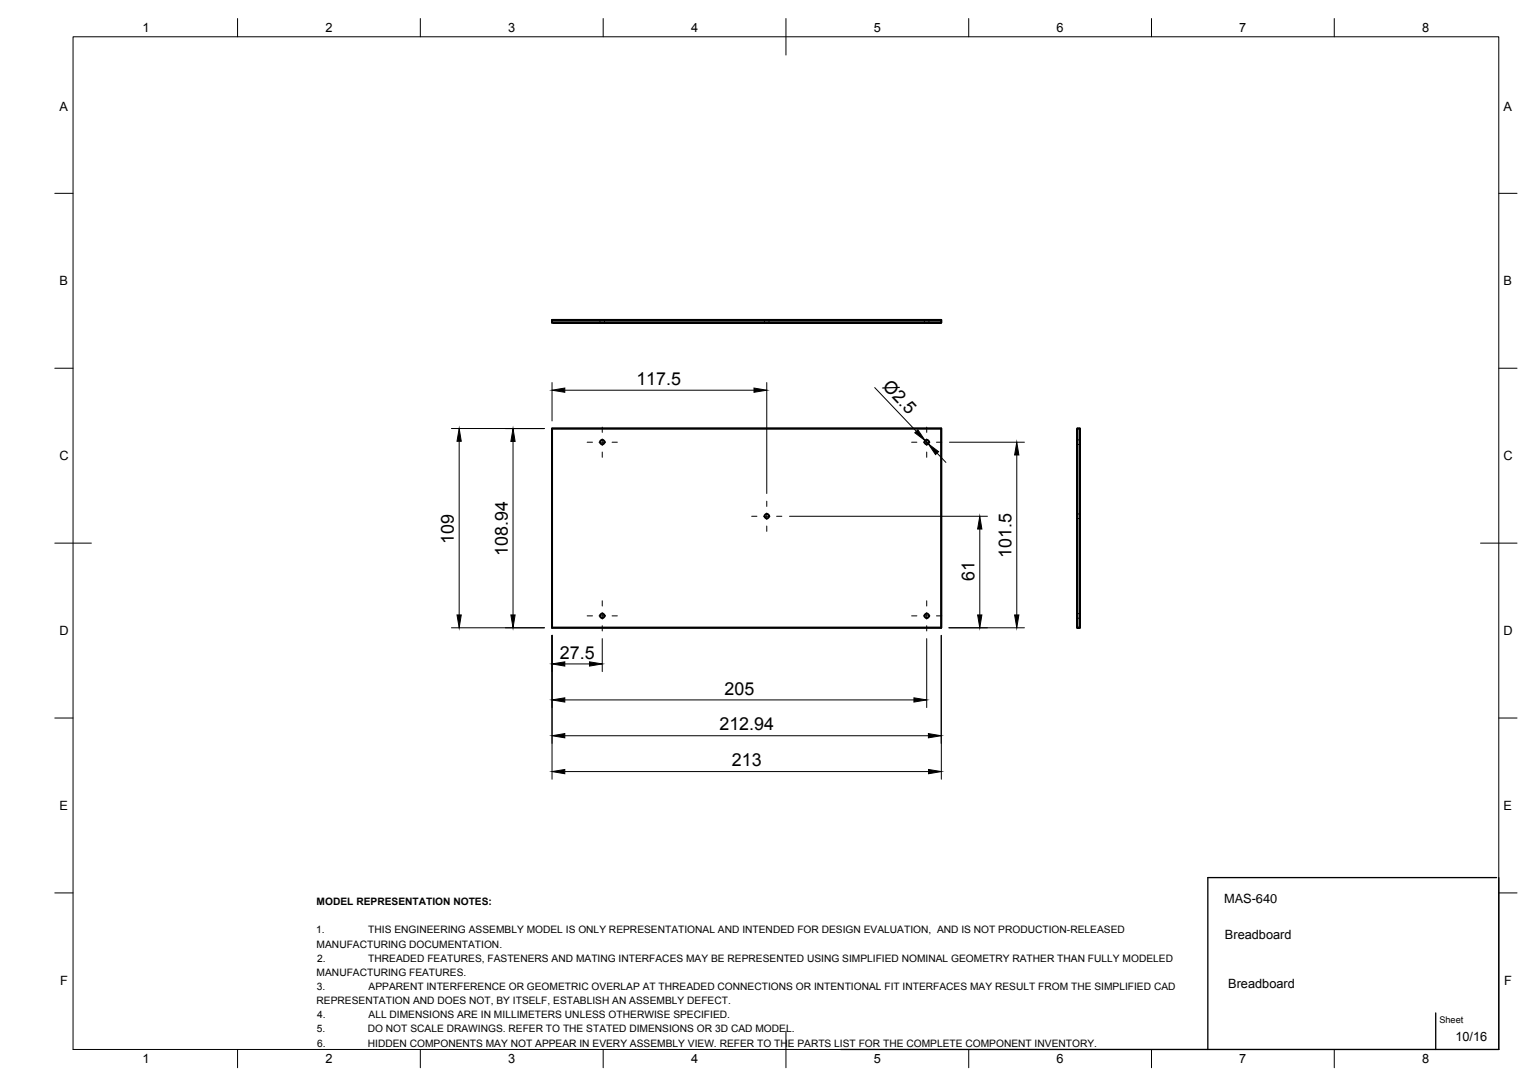
ISO-10303-21;
HEADER;
FILE_DESCRIPTION((''),'2;1');
FILE_NAME('Breadboard.step','2026-10-09T10:33:02-07:00',(''),(''),'','','');
FILE_SCHEMA (('AUTOMOTIVE_DESIGN { 1 0 10303 214 3 1 1 }'));
ENDSEC;
DATA;
#10=MECHANICAL_DESIGN_GEOMETRIC_PRESENTATION_REPRESENTATION('',(#846),#86330);
#822=SHAPE_REPRESENTATION_RELATIONSHIP('SRR','None',#86468,#834) ;
#834=ADVANCED_BREP_SHAPE_REPRESENTATION('',(#858),#86322) ;
#846=STYLED_ITEM('',(#86584),#858) ;
#858=MANIFOLD_SOLID_BREP('Body1',#32645) ;
#1175=FACE_BOUND('',#6134,.T.) ;
#1176=FACE_BOUND('',#6135,.T.) ;
#1177=FACE_BOUND('',#6136,.T.) ;
#1178=FACE_BOUND('',#6137,.T.) ;
#1179=FACE_BOUND('',#6138,.T.) ;
#1180=FACE_BOUND('',#6140,.T.) ;
#1181=FACE_BOUND('',#6141,.T.) ;
#1182=FACE_BOUND('',#6142,.T.) ;
#1183=FACE_BOUND('',#6143,.T.) ;
#1184=FACE_BOUND('',#6144,.T.) ;
#2229=PLANE('',#36344) ;
#2230=PLANE('',#36345) ;
#2231=PLANE('',#36346) ;
#2232=PLANE('',#36347) ;
#2233=PLANE('',#36348) ;
#2234=PLANE('',#36349) ;
#2235=PLANE('',#36350) ;
#2236=PLANE('',#36351) ;
#2237=PLANE('',#36352) ;
#2238=PLANE('',#36353) ;
#2239=PLANE('',#36354) ;
#2240=PLANE('',#36355) ;
#2241=PLANE('',#36356) ;
#2242=PLANE('',#36362) ;
#2243=PLANE('',#36368) ;
#2244=PLANE('',#36369) ;
#2245=PLANE('',#36370) ;
#2246=PLANE('',#36371) ;
#4058=FACE_OUTER_BOUND('',#6121,.T.) ;
#4059=FACE_OUTER_BOUND('',#6122,.T.) ;
#4060=FACE_OUTER_BOUND('',#6123,.T.) ;
#4061=FACE_OUTER_BOUND('',#6124,.T.) ;
#4062=FACE_OUTER_BOUND('',#6125,.T.) ;
#4063=FACE_OUTER_BOUND('',#6126,.T.) ;
#4064=FACE_OUTER_BOUND('',#6127,.T.) ;
#4065=FACE_OUTER_BOUND('',#6128,.T.) ;
#4066=FACE_OUTER_BOUND('',#6129,.T.) ;
#4067=FACE_OUTER_BOUND('',#6130,.T.) ;
#4068=FACE_OUTER_BOUND('',#6131,.T.) ;
#4069=FACE_OUTER_BOUND('',#6132,.T.) ;
#4070=FACE_OUTER_BOUND('',#6133,.T.) ;
#4071=FACE_OUTER_BOUND('',#6139,.T.) ;
#4072=FACE_OUTER_BOUND('',#6145,.T.) ;
#4073=FACE_OUTER_BOUND('',#6146,.T.) ;
#4074=FACE_OUTER_BOUND('',#6147,.T.) ;
#4075=FACE_OUTER_BOUND('',#6148,.T.) ;
#4076=FACE_OUTER_BOUND('',#6149,.T.) ;
#4077=FACE_OUTER_BOUND('',#6150,.T.) ;
#4078=FACE_OUTER_BOUND('',#6151,.T.) ;
#4079=FACE_OUTER_BOUND('',#6152,.T.) ;
#4080=FACE_OUTER_BOUND('',#6153,.T.) ;
#6121=EDGE_LOOP('',(#29412,#29413,#29414,#29415,#29416,#29417)) ;
#6122=EDGE_LOOP('',(#29418,#29419,#29420,#29421,#29422,#29423)) ;
#6123=EDGE_LOOP('',(#29424,#29425,#29426,#29427,#29428,#29429)) ;
#6124=EDGE_LOOP('',(#29430,#29431,#29432,#29433)) ;
#6125=EDGE_LOOP('',(#29434,#29435,#29436,#29437,#29438,#29439)) ;
#6126=EDGE_LOOP('',(#29440,#29441,#29442,#29443,#29444,#29445)) ;
#6127=EDGE_LOOP('',(#29446,#29447,#29448,#29449,#29450,#29451)) ;
#6128=EDGE_LOOP('',(#29452,#29453,#29454,#29455,#29456,#29457)) ;
#6129=EDGE_LOOP('',(#29458,#29459,#29460,#29461)) ;
#6130=EDGE_LOOP('',(#29462,#29463,#29464,#29465,#29466,#29467)) ;
#6131=EDGE_LOOP('',(#29468,#29469,#29470,#29471,#29472,#29473)) ;
#6132=EDGE_LOOP('',(#29474,#29475,#29476,#29477)) ;
#6133=EDGE_LOOP('',(#29478,#29479,#29480,#29481)) ;
#6134=EDGE_LOOP('',(#29482)) ;
#6135=EDGE_LOOP('',(#29483)) ;
#6136=EDGE_LOOP('',(#29484)) ;
#6137=EDGE_LOOP('',(#29485)) ;
#6138=EDGE_LOOP('',(#29486)) ;
#6139=EDGE_LOOP('',(#29487,#29488,#29489,#29490)) ;
#6140=EDGE_LOOP('',(#29491)) ;
#6141=EDGE_LOOP('',(#29492)) ;
#6142=EDGE_LOOP('',(#29493)) ;
#6143=EDGE_LOOP('',(#29494)) ;
#6144=EDGE_LOOP('',(#29495)) ;
#6145=EDGE_LOOP('',(#29496,#29497,#29498,#29499,#29500,#29501)) ;
#6146=EDGE_LOOP('',(#29502,#29503,#29504,#29505)) ;
#6147=EDGE_LOOP('',(#29506,#29507,#29508,#29509,#29510,#29511)) ;
#6148=EDGE_LOOP('',(#29512,#29513,#29514,#29515,#29516,#29517)) ;
#6149=EDGE_LOOP('',(#29518,#29519,#29520,#29521)) ;
#6150=EDGE_LOOP('',(#29522,#29523,#29524,#29525)) ;
#6151=EDGE_LOOP('',(#29526,#29527,#29528,#29529)) ;
#6152=EDGE_LOOP('',(#29530,#29531,#29532,#29533)) ;
#6153=EDGE_LOOP('',(#29534,#29535,#29536,#29537)) ;
#8429=LINE('',#81667,#10748) ;
#8430=LINE('',#81669,#10749) ;
#8431=LINE('',#81671,#10750) ;
#8432=LINE('',#81673,#10751) ;
#8433=LINE('',#81675,#10752) ;
#8434=LINE('',#81676,#10753) ;
#8435=LINE('',#81679,#10754) ;
#8436=LINE('',#81681,#10755) ;
#8437=LINE('',#81683,#10756) ;
#8438=LINE('',#81685,#10757) ;
#8439=LINE('',#81686,#10758) ;
#8440=LINE('',#81689,#10759) ;
#8441=LINE('',#81691,#10760) ;
#8442=LINE('',#81693,#10761) ;
#8443=LINE('',#81694,#10762) ;
#8444=LINE('',#81697,#10763) ;
#8445=LINE('',#81698,#10764) ;
#8446=LINE('',#81702,#10765) ;
#8447=LINE('',#81704,#10766) ;
#8448=LINE('',#81705,#10767) ;
#8449=LINE('',#81706,#10768) ;
#8450=LINE('',#81709,#10769) ;
#8451=LINE('',#81711,#10770) ;
#8452=LINE('',#81713,#10771) ;
#8453=LINE('',#81714,#10772) ;
#8454=LINE('',#81718,#10773) ;
#8455=LINE('',#81720,#10774) ;
#8456=LINE('',#81721,#10775) ;
#8457=LINE('',#81723,#10776) ;
#8458=LINE('',#81724,#10777) ;
#8459=LINE('',#81727,#10778) ;
#8460=LINE('',#81728,#10779) ;
#8461=LINE('',#81729,#10780) ;
#8462=LINE('',#81732,#10781) ;
#8463=LINE('',#81733,#10782) ;
#8464=LINE('',#81736,#10783) ;
#8465=LINE('',#81738,#10784) ;
#8466=LINE('',#81740,#10785) ;
#8467=LINE('',#81741,#10786) ;
#8468=LINE('',#81744,#10787) ;
#8469=LINE('',#81745,#10788) ;
#8470=LINE('',#81748,#10789) ;
#8471=LINE('',#81760,#10790) ;
#8472=LINE('',#81773,#10791) ;
#8473=LINE('',#81774,#10792) ;
#8474=LINE('',#81777,#10793) ;
#8475=LINE('',#81778,#10794) ;
#8476=LINE('',#81780,#10795) ;
#8477=LINE('',#81783,#10796) ;
#8478=LINE('',#81785,#10797) ;
#8479=LINE('',#81787,#10798) ;
#8480=LINE('',#81789,#10799) ;
#8481=LINE('',#81791,#10800) ;
#10748=VECTOR('',#45865,10.) ;
#10749=VECTOR('',#45866,10.) ;
#10750=VECTOR('',#45867,10.) ;
#10751=VECTOR('',#45868,9.99999999999998) ;
#10752=VECTOR('',#45869,10.) ;
#10753=VECTOR('',#45870,10.) ;
#10754=VECTOR('',#45873,10.) ;
#10755=VECTOR('',#45874,10.) ;
#10756=VECTOR('',#45875,10.) ;
#10757=VECTOR('',#45876,10.) ;
#10758=VECTOR('',#45877,10.) ;
#10759=VECTOR('',#45880,10.) ;
#10760=VECTOR('',#45881,10.) ;
#10761=VECTOR('',#45882,10.) ;
#10762=VECTOR('',#45883,10.) ;
#10763=VECTOR('',#45886,10.) ;
#10764=VECTOR('',#45887,10.) ;
#10765=VECTOR('',#45890,10.) ;
#10766=VECTOR('',#45891,10.) ;
#10767=VECTOR('',#45892,10.) ;
#10768=VECTOR('',#45893,10.) ;
#10769=VECTOR('',#45896,10.) ;
#10770=VECTOR('',#45897,10.) ;
#10771=VECTOR('',#45898,10.) ;
#10772=VECTOR('',#45899,10.) ;
#10773=VECTOR('',#45902,10.) ;
#10774=VECTOR('',#45903,10.) ;
#10775=VECTOR('',#45904,10.) ;
#10776=VECTOR('',#45905,10.) ;
#10777=VECTOR('',#45906,10.) ;
#10778=VECTOR('',#45909,10.) ;
#10779=VECTOR('',#45910,10.) ;
#10780=VECTOR('',#45911,10.) ;
#10781=VECTOR('',#45914,10.) ;
#10782=VECTOR('',#45915,10.) ;
#10783=VECTOR('',#45918,10.) ;
#10784=VECTOR('',#45919,10.) ;
#10785=VECTOR('',#45920,10.) ;
#10786=VECTOR('',#45921,10.) ;
#10787=VECTOR('',#45924,10.) ;
#10788=VECTOR('',#45925,10.) ;
#10789=VECTOR('',#45930,10.) ;
#10790=VECTOR('',#45943,10.) ;
#10791=VECTOR('',#45956,10.) ;
#10792=VECTOR('',#45957,10.) ;
#10793=VECTOR('',#45960,10.) ;
#10794=VECTOR('',#45961,10.) ;
#10795=VECTOR('',#45964,10.) ;
#10796=VECTOR('',#45969,1.25) ;
#10797=VECTOR('',#45972,1.25) ;
#10798=VECTOR('',#45975,1.25) ;
#10799=VECTOR('',#45978,1.25) ;
#10800=VECTOR('',#45981,1.25) ;
#12609=CIRCLE('',#36357,1.25) ;
#12610=CIRCLE('',#36358,1.25) ;
#12611=CIRCLE('',#36359,1.25) ;
#12612=CIRCLE('',#36360,1.25) ;
#12613=CIRCLE('',#36361,1.25) ;
#12614=CIRCLE('',#36363,1.25) ;
#12615=CIRCLE('',#36364,1.25) ;
#12616=CIRCLE('',#36365,1.25) ;
#12617=CIRCLE('',#36366,1.25) ;
#12618=CIRCLE('',#36367,1.25) ;
#15418=VERTEX_POINT('',#81665) ;
#15419=VERTEX_POINT('',#81666) ;
#15420=VERTEX_POINT('',#81668) ;
#15421=VERTEX_POINT('',#81670) ;
#15422=VERTEX_POINT('',#81672) ;
#15423=VERTEX_POINT('',#81674) ;
#15424=VERTEX_POINT('',#81678) ;
#15425=VERTEX_POINT('',#81680) ;
#15426=VERTEX_POINT('',#81682) ;
#15427=VERTEX_POINT('',#81684) ;
#15428=VERTEX_POINT('',#81688) ;
#15429=VERTEX_POINT('',#81690) ;
#15430=VERTEX_POINT('',#81692) ;
#15431=VERTEX_POINT('',#81696) ;
#15432=VERTEX_POINT('',#81700) ;
#15433=VERTEX_POINT('',#81701) ;
#15434=VERTEX_POINT('',#81703) ;
#15435=VERTEX_POINT('',#81708) ;
#15436=VERTEX_POINT('',#81710) ;
#15437=VERTEX_POINT('',#81712) ;
#15438=VERTEX_POINT('',#81716) ;
#15439=VERTEX_POINT('',#81717) ;
#15440=VERTEX_POINT('',#81719) ;
#15441=VERTEX_POINT('',#81722) ;
#15442=VERTEX_POINT('',#81726) ;
#15443=VERTEX_POINT('',#81731) ;
#15444=VERTEX_POINT('',#81735) ;
#15445=VERTEX_POINT('',#81737) ;
#15446=VERTEX_POINT('',#81739) ;
#15447=VERTEX_POINT('',#81743) ;
#15448=VERTEX_POINT('',#81749) ;
#15449=VERTEX_POINT('',#81751) ;
#15450=VERTEX_POINT('',#81753) ;
#15451=VERTEX_POINT('',#81755) ;
#15452=VERTEX_POINT('',#81757) ;
#15453=VERTEX_POINT('',#81761) ;
#15454=VERTEX_POINT('',#81763) ;
#15455=VERTEX_POINT('',#81765) ;
#15456=VERTEX_POINT('',#81767) ;
#15457=VERTEX_POINT('',#81769) ;
#15458=VERTEX_POINT('',#81772) ;
#15459=VERTEX_POINT('',#81776) ;
#20112=EDGE_CURVE('',#15418,#15419,#8429,.T.) ;
#20113=EDGE_CURVE('',#15419,#15420,#8430,.T.) ;
#20114=EDGE_CURVE('',#15420,#15421,#8431,.T.) ;
#20115=EDGE_CURVE('',#15421,#15422,#8432,.T.) ;
#20116=EDGE_CURVE('',#15422,#15423,#8433,.T.) ;
#20117=EDGE_CURVE('',#15423,#15418,#8434,.T.) ;
#20118=EDGE_CURVE('',#15424,#15421,#8435,.T.) ;
#20119=EDGE_CURVE('',#15424,#15425,#8436,.T.) ;
#20120=EDGE_CURVE('',#15426,#15425,#8437,.T.) ;
#20121=EDGE_CURVE('',#15427,#15426,#8438,.T.) ;
#20122=EDGE_CURVE('',#15427,#15422,#8439,.T.) ;
#20123=EDGE_CURVE('',#15420,#15428,#8440,.T.) ;
#20124=EDGE_CURVE('',#15429,#15428,#8441,.T.) ;
#20125=EDGE_CURVE('',#15429,#15430,#8442,.T.) ;
#20126=EDGE_CURVE('',#15430,#15424,#8443,.T.) ;
#20127=EDGE_CURVE('',#15431,#15419,#8444,.T.) ;
#20128=EDGE_CURVE('',#15428,#15431,#8445,.T.) ;
#20129=EDGE_CURVE('',#15432,#15433,#8446,.T.) ;
#20130=EDGE_CURVE('',#15433,#15434,#8447,.T.) ;
#20131=EDGE_CURVE('',#15434,#15429,#8448,.T.) ;
#20132=EDGE_CURVE('',#15431,#15432,#8449,.T.) ;
#20133=EDGE_CURVE('',#15434,#15435,#8450,.T.) ;
#20134=EDGE_CURVE('',#15436,#15435,#8451,.T.) ;
#20135=EDGE_CURVE('',#15437,#15436,#8452,.T.) ;
#20136=EDGE_CURVE('',#15437,#15430,#8453,.T.) ;
#20137=EDGE_CURVE('',#15438,#15439,#8454,.T.) ;
#20138=EDGE_CURVE('',#15439,#15440,#8455,.T.) ;
#20139=EDGE_CURVE('',#15440,#15436,#8456,.T.) ;
#20140=EDGE_CURVE('',#15435,#15441,#8457,.T.) ;
#20141=EDGE_CURVE('',#15441,#15438,#8458,.T.) ;
#20142=EDGE_CURVE('',#15440,#15442,#8459,.T.) ;
#20143=EDGE_CURVE('',#15426,#15442,#8460,.T.) ;
#20144=EDGE_CURVE('',#15425,#15437,#8461,.T.) ;
#20145=EDGE_CURVE('',#15443,#15439,#8462,.T.) ;
#20146=EDGE_CURVE('',#15442,#15443,#8463,.T.) ;
#20147=EDGE_CURVE('',#15444,#15438,#8464,.T.) ;
#20148=EDGE_CURVE('',#15444,#15445,#8465,.T.) ;
#20149=EDGE_CURVE('',#15446,#15445,#8466,.T.) ;
#20150=EDGE_CURVE('',#15443,#15446,#8467,.T.) ;
#20151=EDGE_CURVE('',#15446,#15447,#8468,.T.) ;
#20152=EDGE_CURVE('',#15447,#15427,#8469,.T.) ;
#20153=EDGE_CURVE('',#15441,#15433,#8470,.T.) ;
#20154=EDGE_CURVE('',#15448,#15448,#12609,.T.) ;
#20155=EDGE_CURVE('',#15449,#15449,#12610,.T.) ;
#20156=EDGE_CURVE('',#15450,#15450,#12611,.T.) ;
#20157=EDGE_CURVE('',#15451,#15451,#12612,.T.) ;
#20158=EDGE_CURVE('',#15452,#15452,#12613,.T.) ;
#20159=EDGE_CURVE('',#15423,#15447,#8471,.T.) ;
#20160=EDGE_CURVE('',#15453,#15453,#12614,.T.) ;
#20161=EDGE_CURVE('',#15454,#15454,#12615,.T.) ;
#20162=EDGE_CURVE('',#15455,#15455,#12616,.T.) ;
#20163=EDGE_CURVE('',#15456,#15456,#12617,.T.) ;
#20164=EDGE_CURVE('',#15457,#15457,#12618,.T.) ;
#20165=EDGE_CURVE('',#15432,#15458,#8472,.T.) ;
#20166=EDGE_CURVE('',#15458,#15444,#8473,.T.) ;
#20167=EDGE_CURVE('',#15459,#15458,#8474,.T.) ;
#20168=EDGE_CURVE('',#15445,#15459,#8475,.T.) ;
#20169=EDGE_CURVE('',#15459,#15418,#8476,.T.) ;
#20170=EDGE_CURVE('',#15452,#15457,#8477,.T.) ;
#20171=EDGE_CURVE('',#15451,#15456,#8478,.T.) ;
#20172=EDGE_CURVE('',#15450,#15455,#8479,.T.) ;
#20173=EDGE_CURVE('',#15449,#15454,#8480,.T.) ;
#20174=EDGE_CURVE('',#15448,#15453,#8481,.T.) ;
#29412=ORIENTED_EDGE('',*,*,#20112,.T.) ;
#29413=ORIENTED_EDGE('',*,*,#20113,.T.) ;
#29414=ORIENTED_EDGE('',*,*,#20114,.T.) ;
#29415=ORIENTED_EDGE('',*,*,#20115,.T.) ;
#29416=ORIENTED_EDGE('',*,*,#20116,.T.) ;
#29417=ORIENTED_EDGE('',*,*,#20117,.T.) ;
#29418=ORIENTED_EDGE('',*,*,#20115,.F.) ;
#29419=ORIENTED_EDGE('',*,*,#20118,.F.) ;
#29420=ORIENTED_EDGE('',*,*,#20119,.T.) ;
#29421=ORIENTED_EDGE('',*,*,#20120,.F.) ;
#29422=ORIENTED_EDGE('',*,*,#20121,.F.) ;
#29423=ORIENTED_EDGE('',*,*,#20122,.T.) ;
#29424=ORIENTED_EDGE('',*,*,#20114,.F.) ;
#29425=ORIENTED_EDGE('',*,*,#20123,.T.) ;
#29426=ORIENTED_EDGE('',*,*,#20124,.F.) ;
#29427=ORIENTED_EDGE('',*,*,#20125,.T.) ;
#29428=ORIENTED_EDGE('',*,*,#20126,.T.) ;
#29429=ORIENTED_EDGE('',*,*,#20118,.T.) ;
#29430=ORIENTED_EDGE('',*,*,#20113,.F.) ;
#29431=ORIENTED_EDGE('',*,*,#20127,.F.) ;
#29432=ORIENTED_EDGE('',*,*,#20128,.F.) ;
#29433=ORIENTED_EDGE('',*,*,#20123,.F.) ;
#29434=ORIENTED_EDGE('',*,*,#20129,.T.) ;
#29435=ORIENTED_EDGE('',*,*,#20130,.T.) ;
#29436=ORIENTED_EDGE('',*,*,#20131,.T.) ;
#29437=ORIENTED_EDGE('',*,*,#20124,.T.) ;
#29438=ORIENTED_EDGE('',*,*,#20128,.T.) ;
#29439=ORIENTED_EDGE('',*,*,#20132,.T.) ;
#29440=ORIENTED_EDGE('',*,*,#20131,.F.) ;
#29441=ORIENTED_EDGE('',*,*,#20133,.T.) ;
#29442=ORIENTED_EDGE('',*,*,#20134,.F.) ;
#29443=ORIENTED_EDGE('',*,*,#20135,.F.) ;
#29444=ORIENTED_EDGE('',*,*,#20136,.T.) ;
#29445=ORIENTED_EDGE('',*,*,#20125,.F.) ;
#29446=ORIENTED_EDGE('',*,*,#20137,.T.) ;
#29447=ORIENTED_EDGE('',*,*,#20138,.T.) ;
#29448=ORIENTED_EDGE('',*,*,#20139,.T.) ;
#29449=ORIENTED_EDGE('',*,*,#20134,.T.) ;
#29450=ORIENTED_EDGE('',*,*,#20140,.T.) ;
#29451=ORIENTED_EDGE('',*,*,#20141,.T.) ;
#29452=ORIENTED_EDGE('',*,*,#20139,.F.) ;
#29453=ORIENTED_EDGE('',*,*,#20142,.T.) ;
#29454=ORIENTED_EDGE('',*,*,#20143,.F.) ;
#29455=ORIENTED_EDGE('',*,*,#20120,.T.) ;
#29456=ORIENTED_EDGE('',*,*,#20144,.T.) ;
#29457=ORIENTED_EDGE('',*,*,#20135,.T.) ;
#29458=ORIENTED_EDGE('',*,*,#20138,.F.) ;
#29459=ORIENTED_EDGE('',*,*,#20145,.F.) ;
#29460=ORIENTED_EDGE('',*,*,#20146,.F.) ;
#29461=ORIENTED_EDGE('',*,*,#20142,.F.) ;
#29462=ORIENTED_EDGE('',*,*,#20137,.F.) ;
#29463=ORIENTED_EDGE('',*,*,#20147,.F.) ;
#29464=ORIENTED_EDGE('',*,*,#20148,.T.) ;
#29465=ORIENTED_EDGE('',*,*,#20149,.F.) ;
#29466=ORIENTED_EDGE('',*,*,#20150,.F.) ;
#29467=ORIENTED_EDGE('',*,*,#20145,.T.) ;
#29468=ORIENTED_EDGE('',*,*,#20143,.T.) ;
#29469=ORIENTED_EDGE('',*,*,#20146,.T.) ;
#29470=ORIENTED_EDGE('',*,*,#20150,.T.) ;
#29471=ORIENTED_EDGE('',*,*,#20151,.T.) ;
#29472=ORIENTED_EDGE('',*,*,#20152,.T.) ;
#29473=ORIENTED_EDGE('',*,*,#20121,.T.) ;
#29474=ORIENTED_EDGE('',*,*,#20144,.F.) ;
#29475=ORIENTED_EDGE('',*,*,#20119,.F.) ;
#29476=ORIENTED_EDGE('',*,*,#20126,.F.) ;
#29477=ORIENTED_EDGE('',*,*,#20136,.F.) ;
#29478=ORIENTED_EDGE('',*,*,#20130,.F.) ;
#29479=ORIENTED_EDGE('',*,*,#20153,.F.) ;
#29480=ORIENTED_EDGE('',*,*,#20140,.F.) ;
#29481=ORIENTED_EDGE('',*,*,#20133,.F.) ;
#29482=ORIENTED_EDGE('',*,*,#20154,.F.) ;
#29483=ORIENTED_EDGE('',*,*,#20155,.F.) ;
#29484=ORIENTED_EDGE('',*,*,#20156,.F.) ;
#29485=ORIENTED_EDGE('',*,*,#20157,.F.) ;
#29486=ORIENTED_EDGE('',*,*,#20158,.F.) ;
#29487=ORIENTED_EDGE('',*,*,#20116,.F.) ;
#29488=ORIENTED_EDGE('',*,*,#20122,.F.) ;
#29489=ORIENTED_EDGE('',*,*,#20152,.F.) ;
#29490=ORIENTED_EDGE('',*,*,#20159,.F.) ;
#29491=ORIENTED_EDGE('',*,*,#20160,.F.) ;
#29492=ORIENTED_EDGE('',*,*,#20161,.F.) ;
#29493=ORIENTED_EDGE('',*,*,#20162,.F.) ;
#29494=ORIENTED_EDGE('',*,*,#20163,.F.) ;
#29495=ORIENTED_EDGE('',*,*,#20164,.F.) ;
#29496=ORIENTED_EDGE('',*,*,#20129,.F.) ;
#29497=ORIENTED_EDGE('',*,*,#20165,.T.) ;
#29498=ORIENTED_EDGE('',*,*,#20166,.T.) ;
#29499=ORIENTED_EDGE('',*,*,#20147,.T.) ;
#29500=ORIENTED_EDGE('',*,*,#20141,.F.) ;
#29501=ORIENTED_EDGE('',*,*,#20153,.T.) ;
#29502=ORIENTED_EDGE('',*,*,#20166,.F.) ;
#29503=ORIENTED_EDGE('',*,*,#20167,.F.) ;
#29504=ORIENTED_EDGE('',*,*,#20168,.F.) ;
#29505=ORIENTED_EDGE('',*,*,#20148,.F.) ;
#29506=ORIENTED_EDGE('',*,*,#20117,.F.) ;
#29507=ORIENTED_EDGE('',*,*,#20159,.T.) ;
#29508=ORIENTED_EDGE('',*,*,#20151,.F.) ;
#29509=ORIENTED_EDGE('',*,*,#20149,.T.) ;
#29510=ORIENTED_EDGE('',*,*,#20168,.T.) ;
#29511=ORIENTED_EDGE('',*,*,#20169,.T.) ;
#29512=ORIENTED_EDGE('',*,*,#20112,.F.) ;
#29513=ORIENTED_EDGE('',*,*,#20169,.F.) ;
#29514=ORIENTED_EDGE('',*,*,#20167,.T.) ;
#29515=ORIENTED_EDGE('',*,*,#20165,.F.) ;
#29516=ORIENTED_EDGE('',*,*,#20132,.F.) ;
#29517=ORIENTED_EDGE('',*,*,#20127,.T.) ;
#29518=ORIENTED_EDGE('',*,*,#20158,.T.) ;
#29519=ORIENTED_EDGE('',*,*,#20170,.T.) ;
#29520=ORIENTED_EDGE('',*,*,#20164,.T.) ;
#29521=ORIENTED_EDGE('',*,*,#20170,.F.) ;
#29522=ORIENTED_EDGE('',*,*,#20157,.T.) ;
#29523=ORIENTED_EDGE('',*,*,#20171,.T.) ;
#29524=ORIENTED_EDGE('',*,*,#20163,.T.) ;
#29525=ORIENTED_EDGE('',*,*,#20171,.F.) ;
#29526=ORIENTED_EDGE('',*,*,#20156,.T.) ;
#29527=ORIENTED_EDGE('',*,*,#20172,.T.) ;
#29528=ORIENTED_EDGE('',*,*,#20162,.T.) ;
#29529=ORIENTED_EDGE('',*,*,#20172,.F.) ;
#29530=ORIENTED_EDGE('',*,*,#20155,.T.) ;
#29531=ORIENTED_EDGE('',*,*,#20173,.T.) ;
#29532=ORIENTED_EDGE('',*,*,#20161,.T.) ;
#29533=ORIENTED_EDGE('',*,*,#20173,.F.) ;
#29534=ORIENTED_EDGE('',*,*,#20154,.T.) ;
#29535=ORIENTED_EDGE('',*,*,#20174,.T.) ;
#29536=ORIENTED_EDGE('',*,*,#20160,.T.) ;
#29537=ORIENTED_EDGE('',*,*,#20174,.F.) ;
#30707=CYLINDRICAL_SURFACE('',#36372,1.25) ;
#30708=CYLINDRICAL_SURFACE('',#36373,1.25) ;
#30709=CYLINDRICAL_SURFACE('',#36374,1.25) ;
#30710=CYLINDRICAL_SURFACE('',#36375,1.25) ;
#30711=CYLINDRICAL_SURFACE('',#36376,1.25) ;
#32537=ADVANCED_FACE('',(#4058),#2229,.T.) ;
#32538=ADVANCED_FACE('',(#4059),#2230,.T.) ;
#32539=ADVANCED_FACE('',(#4060),#2231,.T.) ;
#32540=ADVANCED_FACE('',(#4061),#2232,.T.) ;
#32541=ADVANCED_FACE('',(#4062),#2233,.T.) ;
#32542=ADVANCED_FACE('',(#4063),#2234,.T.) ;
#32543=ADVANCED_FACE('',(#4064),#2235,.T.) ;
#32544=ADVANCED_FACE('',(#4065),#2236,.T.) ;
#32545=ADVANCED_FACE('',(#4066),#2237,.T.) ;
#32546=ADVANCED_FACE('',(#4067),#2238,.T.) ;
#32547=ADVANCED_FACE('',(#4068),#2239,.T.) ;
#32548=ADVANCED_FACE('',(#4069),#2240,.T.) ;
#32549=ADVANCED_FACE('',(#4070,#1175,#1176,#1177,#1178,#1179),#2241,.T.) ;
#32550=ADVANCED_FACE('',(#4071,#1180,#1181,#1182,#1183,#1184),#2242,.T.) ;
#32551=ADVANCED_FACE('',(#4072),#2243,.T.) ;
#32552=ADVANCED_FACE('',(#4073),#2244,.F.) ;
#32553=ADVANCED_FACE('',(#4074),#2245,.T.) ;
#32554=ADVANCED_FACE('',(#4075),#2246,.T.) ;
#32555=ADVANCED_FACE('',(#4076),#30707,.F.) ;
#32556=ADVANCED_FACE('',(#4077),#30708,.F.) ;
#32557=ADVANCED_FACE('',(#4078),#30709,.F.) ;
#32558=ADVANCED_FACE('',(#4079),#30710,.F.) ;
#32559=ADVANCED_FACE('',(#4080),#30711,.F.) ;
#32645=CLOSED_SHELL('',(#32537,#32538,#32539,#32540,#32541,#32542,#32543,
#32544,#32545,#32546,#32547,#32548,#32549,#32550,#32551,#32552,#32553,#32554,
#32555,#32556,#32557,#32558,#32559)) ;
#36343=AXIS2_PLACEMENT_3D('',#81663,#45861,#45862) ;
#36344=AXIS2_PLACEMENT_3D('',#81664,#45863,#45864) ;
#36345=AXIS2_PLACEMENT_3D('',#81677,#45871,#45872) ;
#36346=AXIS2_PLACEMENT_3D('',#81687,#45878,#45879) ;
#36347=AXIS2_PLACEMENT_3D('',#81695,#45884,#45885) ;
#36348=AXIS2_PLACEMENT_3D('',#81699,#45888,#45889) ;
#36349=AXIS2_PLACEMENT_3D('',#81707,#45894,#45895) ;
#36350=AXIS2_PLACEMENT_3D('',#81715,#45900,#45901) ;
#36351=AXIS2_PLACEMENT_3D('',#81725,#45907,#45908) ;
#36352=AXIS2_PLACEMENT_3D('',#81730,#45912,#45913) ;
#36353=AXIS2_PLACEMENT_3D('',#81734,#45916,#45917) ;
#36354=AXIS2_PLACEMENT_3D('',#81742,#45922,#45923) ;
#36355=AXIS2_PLACEMENT_3D('',#81746,#45926,#45927) ;
#36356=AXIS2_PLACEMENT_3D('',#81747,#45928,#45929) ;
#36357=AXIS2_PLACEMENT_3D('',#81750,#45931,#45932) ;
#36358=AXIS2_PLACEMENT_3D('',#81752,#45933,#45934) ;
#36359=AXIS2_PLACEMENT_3D('',#81754,#45935,#45936) ;
#36360=AXIS2_PLACEMENT_3D('',#81756,#45937,#45938) ;
#36361=AXIS2_PLACEMENT_3D('',#81758,#45939,#45940) ;
#36362=AXIS2_PLACEMENT_3D('',#81759,#45941,#45942) ;
#36363=AXIS2_PLACEMENT_3D('',#81762,#45944,#45945) ;
#36364=AXIS2_PLACEMENT_3D('',#81764,#45946,#45947) ;
#36365=AXIS2_PLACEMENT_3D('',#81766,#45948,#45949) ;
#36366=AXIS2_PLACEMENT_3D('',#81768,#45950,#45951) ;
#36367=AXIS2_PLACEMENT_3D('',#81770,#45952,#45953) ;
#36368=AXIS2_PLACEMENT_3D('',#81771,#45954,#45955) ;
#36369=AXIS2_PLACEMENT_3D('',#81775,#45958,#45959) ;
#36370=AXIS2_PLACEMENT_3D('',#81779,#45962,#45963) ;
#36371=AXIS2_PLACEMENT_3D('',#81781,#45965,#45966) ;
#36372=AXIS2_PLACEMENT_3D('',#81782,#45967,#45968) ;
#36373=AXIS2_PLACEMENT_3D('',#81784,#45970,#45971) ;
#36374=AXIS2_PLACEMENT_3D('',#81786,#45973,#45974) ;
#36375=AXIS2_PLACEMENT_3D('',#81788,#45976,#45977) ;
#36376=AXIS2_PLACEMENT_3D('',#81790,#45979,#45980) ;
#45861=DIRECTION('axis',(0.,0.,1.)) ;
#45862=DIRECTION('refdir',(1.,0.,0.)) ;
#45863=DIRECTION('center_axis',(-3.21164817626321E-14,0.707106781183433,
-0.707106781189663)) ;
#45864=DIRECTION('ref_axis',(-1.,4.59435859315612E-29,4.54195640842224E-14)) ;
#45865=DIRECTION('',(-0.577350269185717,-0.577350269194137,-0.577350269189023)) ;
#45866=DIRECTION('',(-1.,-4.54195640846222E-14,4.43134223659454E-28)) ;
#45867=DIRECTION('',(-0.577350269188067,0.577350269192936,0.577350269187875)) ;
#45868=DIRECTION('',(0.57735026919122,0.577350269191385,0.577350269186272)) ;
#45869=DIRECTION('',(1.,4.54195640846222E-14,-4.43134223659454E-28)) ;
#45870=DIRECTION('',(0.577350269190983,-0.577350269191477,-0.577350269186417)) ;
#45871=DIRECTION('center_axis',(-0.707106781186648,0.707106781186447,-2.17344707950985E-15)) ;
#45872=DIRECTION('ref_axis',(-3.07371833694259E-15,-1.89978378844695E-30,
1.)) ;
#45873=DIRECTION('',(0.577350269189617,0.577350269189779,-0.577350269189481)) ;
#45874=DIRECTION('',(3.03527276676558E-28,3.07371833694377E-15,1.)) ;
#45875=DIRECTION('',(-0.577350269189562,-0.577350269189728,-0.577350269189587)) ;
#45876=DIRECTION('',(-0.577350269187503,-0.577350269187665,0.57735026919371)) ;
#45877=DIRECTION('',(-3.03527276676558E-28,-3.07371833694377E-15,-1.)) ;
#45878=DIRECTION('center_axis',(-0.707106781186447,-3.42899288422795E-14,
-0.707106781186648)) ;
#45879=DIRECTION('ref_axis',(-0.707106781186648,-5.24209240922293E-31,0.707106781186447)) ;
#45880=DIRECTION('',(4.54195640846222E-14,-1.,3.07371833694377E-15)) ;
#45881=DIRECTION('',(0.577350269189872,0.57735026918927,-0.577350269189736)) ;
#45882=DIRECTION('',(-0.577350269189744,0.577350269189582,0.577350269189552)) ;
#45883=DIRECTION('',(-4.54195640846222E-14,1.,-3.07371833694377E-15)) ;
#45884=DIRECTION('center_axis',(-3.03527276676558E-28,-3.07371833694377E-15,
-1.)) ;
#45885=DIRECTION('ref_axis',(-4.54195640846222E-14,1.,-3.07371833694377E-15)) ;
#45886=DIRECTION('',(-4.54195640846222E-14,1.,-3.07371833694377E-15)) ;
#45887=DIRECTION('',(1.,4.54195640846222E-14,-4.43134223659454E-28)) ;
#45888=DIRECTION('center_axis',(3.21164817627867E-14,-0.707106781186849,
-0.707106781186246)) ;
#45889=DIRECTION('ref_axis',(-1.,1.22805031005106E-29,-4.54195640846605E-14)) ;
#45890=DIRECTION('',(-0.577350269186846,-0.577350269190783,0.577350269191249)) ;
#45891=DIRECTION('',(-1.,-4.54195640846222E-14,4.43134223659454E-28)) ;
#45892=DIRECTION('',(-0.577350269189563,0.577350269189398,-0.577350269189916)) ;
#45893=DIRECTION('',(0.577350269187627,-0.577350269190366,0.577350269190884)) ;
#45894=DIRECTION('center_axis',(-0.707106781186447,-0.707106781186648,2.1734470795109E-15)) ;
#45895=DIRECTION('ref_axis',(3.07371833694495E-15,-2.57298801481783E-30,
1.)) ;
#45896=DIRECTION('',(3.03527276676558E-28,3.07371833694377E-15,1.)) ;
#45897=DIRECTION('',(0.577350269189561,-0.577350269189399,-0.577350269189917)) ;
#45898=DIRECTION('',(0.577350269189689,-0.577350269189523,0.577350269189665)) ;
#45899=DIRECTION('',(-3.03527276676558E-28,-3.07371833694377E-15,-1.)) ;
#45900=DIRECTION('center_axis',(3.21164817627873E-14,-0.707106781186849,
0.707106781186246)) ;
#45901=DIRECTION('ref_axis',(1.,-5.21959547942856E-29,-4.54195640846614E-14)) ;
#45902=DIRECTION('',(-0.577350269188176,0.577350269190091,0.57735026919061)) ;
#45903=DIRECTION('',(-1.,-4.54195640846222E-14,4.43134223659454E-28)) ;
#45904=DIRECTION('',(-0.577350269189765,-0.577350269189323,-0.577350269189789)) ;
#45905=DIRECTION('',(1.,4.54195640846222E-14,-4.43134223659454E-28)) ;
#45906=DIRECTION('',(0.577350269186844,0.577350269190784,0.57735026919125)) ;
#45907=DIRECTION('center_axis',(-0.707106781186548,-2.9943034683263E-14,
0.707106781186548)) ;
#45908=DIRECTION('ref_axis',(0.707106781186548,4.34801313340064E-31,0.707106781186548)) ;
#45909=DIRECTION('',(-4.54195640846222E-14,1.,-3.07371833694377E-15)) ;
#45910=DIRECTION('',(0.577350269191675,-0.577350269185553,0.57735026919165)) ;
#45911=DIRECTION('',(4.54195640846222E-14,-1.,3.07371833694377E-15)) ;
#45912=DIRECTION('center_axis',(3.03527276676558E-28,3.07371833694377E-15,
1.)) ;
#45913=DIRECTION('ref_axis',(4.54195640846222E-14,-1.,3.07371833694377E-15)) ;
#45914=DIRECTION('',(4.54195640846222E-14,-1.,3.07371833694377E-15)) ;
#45915=DIRECTION('',(1.,4.54195640846222E-14,-4.43134223659454E-28)) ;
#45916=DIRECTION('center_axis',(0.707106781188055,3.42899288423475E-14,
0.70710678118504)) ;
#45917=DIRECTION('ref_axis',(0.70710678118504,-2.67373424278474E-31,-0.707106781188055)) ;
#45918=DIRECTION('',(-0.577350269187484,-0.57735026919142,0.577350269189973)) ;
#45919=DIRECTION('',(-4.54195640846222E-14,1.,-3.07371833694377E-15)) ;
#45920=DIRECTION('',(0.57735026918865,-0.577350269189144,-0.577350269191083)) ;
#45921=DIRECTION('',(0.577350269189981,0.577350269186425,-0.577350269192471)) ;
#45922=DIRECTION('center_axis',(-3.21164817629419E-14,0.707106781190265,
0.70710678118283)) ;
#45923=DIRECTION('ref_axis',(1.,-2.00665671353E-30,4.54195640850994E-14)) ;
#45924=DIRECTION('',(-0.577350269187266,0.577350269187757,-0.577350269193854)) ;
#45925=DIRECTION('',(-1.,-4.54195640846222E-14,4.43134223659454E-28)) ;
#45926=DIRECTION('center_axis',(-1.,-4.54195640846222E-14,4.43134223659454E-28)) ;
#45927=DIRECTION('ref_axis',(4.54195640846222E-14,-1.,3.07371833694377E-15)) ;
#45928=DIRECTION('center_axis',(4.54195640846222E-14,-1.,3.07371833694377E-15)) ;
#45929=DIRECTION('ref_axis',(-3.03527276676558E-28,-3.07371833694377E-15,
-1.)) ;
#45930=DIRECTION('',(-6.99265107823647E-28,-3.07371833694377E-15,-1.)) ;
#45931=DIRECTION('center_axis',(4.54195640846222E-14,-1.,3.07371833694377E-15)) ;
#45932=DIRECTION('ref_axis',(6.81575822110954E-28,3.07371833694377E-15,
1.)) ;
#45933=DIRECTION('center_axis',(4.54195640846222E-14,-1.,3.07371833694377E-15)) ;
#45934=DIRECTION('ref_axis',(6.81575822110954E-28,3.07371833694377E-15,
1.)) ;
#45935=DIRECTION('center_axis',(4.54195640846222E-14,-1.,3.07371833694377E-15)) ;
#45936=DIRECTION('ref_axis',(6.81575822110954E-28,3.07371833694377E-15,
1.)) ;
#45937=DIRECTION('center_axis',(4.54195640846222E-14,-1.,3.07371833694377E-15)) ;
#45938=DIRECTION('ref_axis',(6.81575822110954E-28,3.07371833694377E-15,
1.)) ;
#45939=DIRECTION('center_axis',(4.54195640846222E-14,-1.,3.07371833694377E-15)) ;
#45940=DIRECTION('ref_axis',(6.81575822110954E-28,3.07371833694377E-15,
1.)) ;
#45941=DIRECTION('center_axis',(-4.54195640846222E-14,1.,-3.07371833694377E-15)) ;
#45942=DIRECTION('ref_axis',(3.03527276676558E-28,3.07371833694377E-15,
1.)) ;
#45943=DIRECTION('',(6.99265107823647E-28,3.07371833694377E-15,1.)) ;
#45944=DIRECTION('center_axis',(-4.54195640846222E-14,1.,-3.07371833694377E-15)) ;
#45945=DIRECTION('ref_axis',(6.81575822110954E-28,3.07371833694377E-15,
1.)) ;
#45946=DIRECTION('center_axis',(-4.54195640846222E-14,1.,-3.07371833694377E-15)) ;
#45947=DIRECTION('ref_axis',(6.81575822110954E-28,3.07371833694377E-15,
1.)) ;
#45948=DIRECTION('center_axis',(-4.54195640846222E-14,1.,-3.07371833694377E-15)) ;
#45949=DIRECTION('ref_axis',(6.81575822110954E-28,3.07371833694377E-15,
1.)) ;
#45950=DIRECTION('center_axis',(-4.54195640846222E-14,1.,-3.07371833694377E-15)) ;
#45951=DIRECTION('ref_axis',(6.81575822110954E-28,3.07371833694377E-15,
1.)) ;
#45952=DIRECTION('center_axis',(-4.54195640846222E-14,1.,-3.07371833694377E-15)) ;
#45953=DIRECTION('ref_axis',(6.81575822110954E-28,3.07371833694377E-15,
1.)) ;
#45954=DIRECTION('center_axis',(0.707106781188959,-0.707106781184136,2.17344707950247E-15)) ;
#45955=DIRECTION('ref_axis',(3.07371833692211E-15,3.40932823150776E-30,
-1.)) ;
#45956=DIRECTION('',(0.57735026918721,0.57735026919115,0.577350269190517)) ;
#45957=DIRECTION('',(6.99265107823647E-28,3.07371833694377E-15,1.)) ;
#45958=DIRECTION('center_axis',(-1.,-4.54195640846222E-14,8.38872054806543E-28)) ;
#45959=DIRECTION('ref_axis',(4.54195640846222E-14,-1.,2.90739654572917E-15)) ;
#45960=DIRECTION('',(4.54195640846222E-14,-1.,3.07371833694377E-15)) ;
#45961=DIRECTION('',(-6.99265107823647E-28,-3.07371833694377E-15,-1.)) ;
#45962=DIRECTION('center_axis',(0.707106781186849,0.707106781186246,-2.17344707950995E-15)) ;
#45963=DIRECTION('ref_axis',(-3.07371833694185E-15,-4.33388060696312E-30,
-1.)) ;
#45964=DIRECTION('',(-0.577350269188377,0.577350269188867,-0.577350269191634)) ;
#45965=DIRECTION('center_axis',(0.707106781188557,2.99430346833604E-14,
-0.707106781184538)) ;
#45966=DIRECTION('ref_axis',(-0.707106781184538,-7.37594522657362E-31,-0.707106781188557)) ;
#45967=DIRECTION('center_axis',(-4.54195640846222E-14,1.,-3.07371833694377E-15)) ;
#45968=DIRECTION('ref_axis',(6.81575822110954E-28,3.07371833694377E-15,
1.)) ;
#45969=DIRECTION('',(-4.54195640846222E-14,1.,-3.07371833694377E-15)) ;
#45970=DIRECTION('center_axis',(-4.54195640846222E-14,1.,-3.07371833694377E-15)) ;
#45971=DIRECTION('ref_axis',(6.81575822110954E-28,3.07371833694377E-15,
1.)) ;
#45972=DIRECTION('',(-4.54195640846222E-14,1.,-3.07371833694377E-15)) ;
#45973=DIRECTION('center_axis',(-4.54195640846222E-14,1.,-3.07371833694377E-15)) ;
#45974=DIRECTION('ref_axis',(6.81575822110954E-28,3.07371833694377E-15,
1.)) ;
#45975=DIRECTION('',(-4.54195640846222E-14,1.,-3.07371833694377E-15)) ;
#45976=DIRECTION('center_axis',(-4.54195640846222E-14,1.,-3.07371833694377E-15)) ;
#45977=DIRECTION('ref_axis',(6.81575822110954E-28,3.07371833694377E-15,
1.)) ;
#45978=DIRECTION('',(-4.54195640846222E-14,1.,-3.07371833694377E-15)) ;
#45979=DIRECTION('center_axis',(-4.54195640846222E-14,1.,-3.07371833694377E-15)) ;
#45980=DIRECTION('ref_axis',(6.81575822110954E-28,3.07371833694377E-15,
1.)) ;
#45981=DIRECTION('',(-4.54195640846222E-14,1.,-3.07371833694377E-15)) ;
#81663=CARTESIAN_POINT('',(0.,0.,0.)) ;
#81664=CARTESIAN_POINT('Origin',(337.29203686942,-83.7093863338387,-225.630746738862)) ;
#81665=CARTESIAN_POINT('',(337.26078686942,-83.7093863338386,-225.630746738861)) ;
#81666=CARTESIAN_POINT('',(337.22953686942,-83.7406363338387,-225.661996738861)) ;
#81667=CARTESIAN_POINT('',(336.938011368168,-84.0321618350953,-225.953522240115)) ;
#81668=CARTESIAN_POINT('',(124.35453686942,-83.7406363338483,-225.661996738861)) ;
#81669=CARTESIAN_POINT('',(337.29203686942,-83.7406363338387,-225.661996738861)) ;
#81670=CARTESIAN_POINT('',(124.32328686942,-83.7093863338482,-225.630746738861)) ;
#81671=CARTESIAN_POINT('',(160.479536869229,-119.865636333962,-261.786996738658)) ;
#81672=CARTESIAN_POINT('',(124.35453686942,-83.6781363338483,-225.599496738862)) ;
#81673=CARTESIAN_POINT('',(173.43787020291,-34.5948030003447,-176.516163405793)) ;
#81674=CARTESIAN_POINT('',(337.22953686942,-83.6781363338387,-225.599496738862)) ;
#81675=CARTESIAN_POINT('',(337.29203686942,-83.6781363338387,-225.599496738862)) ;
#81676=CARTESIAN_POINT('',(323.541895704049,-69.9904951684558,-211.911855573599)) ;
#81677=CARTESIAN_POINT('Origin',(124.32328686942,-83.7093863338481,-143.911996738861)) ;
#81678=CARTESIAN_POINT('',(124.29203686942,-83.7406363338483,-225.599496738861)) ;
#81679=CARTESIAN_POINT('',(110.042036869424,-97.9906363338488,-211.349496738868)) ;
#81680=CARTESIAN_POINT('',(124.29203686942,-83.740636333848,-116.724496738861)) ;
#81681=CARTESIAN_POINT('',(124.29203686942,-83.7406363338481,-143.911996738861)) ;
#81682=CARTESIAN_POINT('',(124.32328686942,-83.7093863338482,-116.693246738861)) ;
#81683=CARTESIAN_POINT('',(119.000370202754,-89.0323030005154,-122.016163405527)) ;
#81684=CARTESIAN_POINT('',(124.35453686942,-83.678136333848,-116.724496738862)) ;
#81685=CARTESIAN_POINT('',(164.354536869176,-43.6781363340809,-156.724496739048)) ;
#81686=CARTESIAN_POINT('',(124.35453686942,-83.6781363338481,-143.911996738861)) ;
#81687=CARTESIAN_POINT('Origin',(124.32328686942,-87.6781363338484,-225.630746738861)) ;
#81688=CARTESIAN_POINT('',(124.35453686942,-85.1156363338484,-225.661996738861)) ;
#81689=CARTESIAN_POINT('',(124.35453686942,-87.6781363338484,-225.661996738861)) ;
#81690=CARTESIAN_POINT('',(124.32328686942,-85.1468863338484,-225.630746738861)) ;
#81691=CARTESIAN_POINT('',(159.396203536119,-50.0739696671863,-260.703663405552)) ;
#81692=CARTESIAN_POINT('',(124.29203686942,-85.1156363338484,-225.599496738861)) ;
#81693=CARTESIAN_POINT('',(120.208703536087,-81.0323030005159,-221.516163405529)) ;
#81694=CARTESIAN_POINT('',(124.29203686942,-87.6781363338484,-225.599496738861)) ;
#81695=CARTESIAN_POINT('Origin',(337.29203686942,-83.6781363338387,-225.661996738861)) ;
#81696=CARTESIAN_POINT('',(337.22953686942,-85.1156363338387,-225.661996738861)) ;
#81697=CARTESIAN_POINT('',(337.22953686942,-85.677289341349,-225.661996738861)) ;
#81698=CARTESIAN_POINT('',(337.29203686942,-85.1156363338387,-225.661996738861)) ;
#81699=CARTESIAN_POINT('Origin',(337.29203686942,-85.1468863338387,-225.630746738861)) ;
#81700=CARTESIAN_POINT('',(337.26078686942,-85.1468863338386,-225.630746738861)) ;
#81701=CARTESIAN_POINT('',(337.22953686942,-85.1781363338387,-225.599496738861)) ;
#81702=CARTESIAN_POINT('',(332.625229037348,-89.7824441659428,-220.995188906753)) ;
#81703=CARTESIAN_POINT('',(124.35453686942,-85.1781363338484,-225.599496738861)) ;
#81704=CARTESIAN_POINT('',(337.29203686942,-85.1781363338387,-225.599496738861)) ;
#81705=CARTESIAN_POINT('',(164.354536869413,-125.178136333829,-185.599496738844)) ;
#81706=CARTESIAN_POINT('',(337.354395704005,-85.240495168424,-225.537137904276)) ;
#81707=CARTESIAN_POINT('Origin',(124.32328686942,-85.1468863338483,-198.411996738861)) ;
#81708=CARTESIAN_POINT('',(124.35453686942,-85.178136333848,-116.724496738861)) ;
#81709=CARTESIAN_POINT('',(124.35453686942,-85.1781363338483,-198.411996738861)) ;
#81710=CARTESIAN_POINT('',(124.32328686942,-85.146886333848,-116.693246738861)) ;
#81711=CARTESIAN_POINT('',(173.43787020275,-134.261469667163,-165.807830072221)) ;
#81712=CARTESIAN_POINT('',(124.29203686942,-85.115636333848,-116.724496738861)) ;
#81713=CARTESIAN_POINT('',(111.250370202751,-72.0739696671828,-129.76616340553)) ;
#81714=CARTESIAN_POINT('',(124.29203686942,-85.1156363338483,-198.411996738861)) ;
#81715=CARTESIAN_POINT('Origin',(337.29203686942,-85.1468863338384,-116.693246738861)) ;
#81716=CARTESIAN_POINT('',(337.26078686942,-85.1468863338384,-116.693246738861)) ;
#81717=CARTESIAN_POINT('',(337.22953686942,-85.1156363338384,-116.661996738861)) ;
#81718=CARTESIAN_POINT('',(337.479395704005,-85.3654951684238,-116.911855573447)) ;
#81719=CARTESIAN_POINT('',(124.35453686942,-85.115636333848,-116.661996738861)) ;
#81720=CARTESIAN_POINT('',(337.29203686942,-85.1156363338384,-116.661996738861)) ;
#81721=CARTESIAN_POINT('',(159.271203536106,-50.1989696671892,-81.7453300721742)) ;
#81722=CARTESIAN_POINT('',(337.22953686942,-85.1781363338384,-116.724496738861)) ;
#81723=CARTESIAN_POINT('',(337.29203686942,-85.1781363338384,-116.724496738861)) ;
#81724=CARTESIAN_POINT('',(323.750511368196,-98.6571618351551,-130.203522240189)) ;
#81725=CARTESIAN_POINT('Origin',(124.32328686942,-88.428136333848,-116.693246738861)) ;
#81726=CARTESIAN_POINT('',(124.35453686942,-83.740636333848,-116.661996738861)) ;
#81727=CARTESIAN_POINT('',(124.354536869421,-88.428136333848,-116.661996738861)) ;
#81728=CARTESIAN_POINT('',(160.604536869668,-119.990636333711,-80.4119967386154)) ;
#81729=CARTESIAN_POINT('',(124.29203686942,-88.428136333848,-116.724496738861)) ;
#81730=CARTESIAN_POINT('Origin',(337.29203686942,-85.1781363338384,-116.661996738861)) ;
#81731=CARTESIAN_POINT('',(337.22953686942,-83.7406363338383,-116.661996738861)) ;
#81732=CARTESIAN_POINT('',(337.22953686942,-86.4272893413486,-116.661996738861)) ;
#81733=CARTESIAN_POINT('',(337.29203686942,-83.7406363338383,-116.661996738861)) ;
#81734=CARTESIAN_POINT('Origin',(337.26078686942,-86.4272893413486,-116.693246738861)) ;
#81735=CARTESIAN_POINT('',(337.29203686942,-85.1156363338383,-116.724496738861)) ;
#81736=CARTESIAN_POINT('',(350.562870202711,-71.8448030004564,-129.99533007221)) ;
#81737=CARTESIAN_POINT('',(337.29203686942,-83.7406363338383,-116.724496738861)) ;
#81738=CARTESIAN_POINT('',(337.29203686942,-86.4272893413486,-116.724496738861)) ;
#81739=CARTESIAN_POINT('',(337.26078686942,-83.7093863338386,-116.693246738861)) ;
#81740=CARTESIAN_POINT('',(342.145921205259,-88.5945206696818,-121.578381074721)) ;
#81741=CARTESIAN_POINT('',(336.813011368171,-84.1571618350851,-116.24547123761)) ;
#81742=CARTESIAN_POINT('Origin',(337.29203686942,-83.7093863338383,-116.693246738862)) ;
#81743=CARTESIAN_POINT('',(337.22953686942,-83.6781363338383,-116.724496738862)) ;
#81744=CARTESIAN_POINT('',(332.833844701487,-79.282444165902,-121.120188906845)) ;
#81745=CARTESIAN_POINT('',(337.29203686942,-83.6781363338383,-116.724496738862)) ;
#81746=CARTESIAN_POINT('Origin',(124.292036869421,-91.6781363338482,-171.161996738861)) ;
#81747=CARTESIAN_POINT('Origin',(337.29203686942,-85.1781363338387,-225.661996738861)) ;
#81748=CARTESIAN_POINT('',(337.22953686942,-85.1781363338386,-197.786149746371)) ;
#81749=CARTESIAN_POINT('',(329.29203686942,-85.1781363338387,-125.411996738862)) ;
#81750=CARTESIAN_POINT('Origin',(329.29203686942,-85.1781363338387,-124.161996738862)) ;
#81751=CARTESIAN_POINT('',(151.79203686942,-85.1781363338468,-125.411996738862)) ;
#81752=CARTESIAN_POINT('Origin',(151.79203686942,-85.1781363338468,-124.161996738862)) ;
#81753=CARTESIAN_POINT('',(151.79203686942,-85.1781363338471,-220.411996738862)) ;
#81754=CARTESIAN_POINT('Origin',(151.79203686942,-85.1781363338471,-219.161996738862)) ;
#81755=CARTESIAN_POINT('',(329.29203686942,-85.178136333839,-220.411996738862)) ;
#81756=CARTESIAN_POINT('Origin',(329.29203686942,-85.178136333839,-219.161996738862)) ;
#81757=CARTESIAN_POINT('',(241.79203686942,-85.1781363338428,-165.911996738862)) ;
#81758=CARTESIAN_POINT('Origin',(241.79203686942,-85.1781363338428,-164.661996738862)) ;
#81759=CARTESIAN_POINT('Origin',(337.29203686942,-83.6781363338383,-116.661996738861)) ;
#81760=CARTESIAN_POINT('',(337.22953686942,-83.6781363338384,-143.286149746371)) ;
#81761=CARTESIAN_POINT('',(329.29203686942,-83.6781363338387,-125.411996738862)) ;
#81762=CARTESIAN_POINT('Origin',(329.29203686942,-83.6781363338387,-124.161996738862)) ;
#81763=CARTESIAN_POINT('',(151.79203686942,-83.6781363338468,-125.411996738862)) ;
#81764=CARTESIAN_POINT('Origin',(151.79203686942,-83.6781363338468,-124.161996738862)) ;
#81765=CARTESIAN_POINT('',(151.79203686942,-83.6781363338471,-220.411996738862)) ;
#81766=CARTESIAN_POINT('Origin',(151.79203686942,-83.6781363338471,-219.161996738862)) ;
#81767=CARTESIAN_POINT('',(329.29203686942,-83.678136333839,-220.411996738862)) ;
#81768=CARTESIAN_POINT('Origin',(329.29203686942,-83.678136333839,-219.161996738862)) ;
#81769=CARTESIAN_POINT('',(241.79203686942,-83.6781363338428,-165.911996738862)) ;
#81770=CARTESIAN_POINT('Origin',(241.79203686942,-83.6781363338428,-164.661996738862)) ;
#81771=CARTESIAN_POINT('Origin',(337.26078686942,-85.1468863338386,-197.786149746371)) ;
#81772=CARTESIAN_POINT('',(337.29203686942,-85.1156363338387,-225.599496738861)) ;
#81773=CARTESIAN_POINT('',(341.813152533571,-80.5945206696563,-221.078381074684)) ;
#81774=CARTESIAN_POINT('',(337.29203686942,-85.1156363338386,-197.786149746371)) ;
#81775=CARTESIAN_POINT('Origin',(337.29203686942,-87.6764423488591,-169.91030275388)) ;
#81776=CARTESIAN_POINT('',(337.29203686942,-83.7406363338387,-225.599496738861)) ;
#81777=CARTESIAN_POINT('',(337.29203686942,-85.677289341349,-225.599496738861)) ;
#81778=CARTESIAN_POINT('',(337.29203686942,-83.7406363338384,-143.286149746371)) ;
#81779=CARTESIAN_POINT('Origin',(337.26078686942,-83.7093863338384,-143.286149746371)) ;
#81780=CARTESIAN_POINT('',(351.31287020277,-97.761469667201,-211.578663405432)) ;
#81781=CARTESIAN_POINT('Origin',(337.26078686942,-85.677289341349,-225.630746738861)) ;
#81782=CARTESIAN_POINT('Origin',(241.79203686942,-90.1781363338429,-164.661996738862)) ;
#81783=CARTESIAN_POINT('',(241.79203686942,-90.1781363338429,-165.911996738862)) ;
#81784=CARTESIAN_POINT('Origin',(329.29203686942,-90.1781363338391,-219.161996738862)) ;
#81785=CARTESIAN_POINT('',(329.29203686942,-90.1781363338391,-220.411996738862)) ;
#81786=CARTESIAN_POINT('Origin',(151.79203686942,-90.1781363338472,-219.161996738862)) ;
#81787=CARTESIAN_POINT('',(151.79203686942,-90.1781363338472,-220.411996738862)) ;
#81788=CARTESIAN_POINT('Origin',(151.79203686942,-90.1781363338469,-124.161996738862)) ;
#81789=CARTESIAN_POINT('',(151.79203686942,-90.1781363338469,-125.411996738862)) ;
#81790=CARTESIAN_POINT('Origin',(329.29203686942,-90.1781363338388,-124.161996738862)) ;
#81791=CARTESIAN_POINT('',(329.29203686942,-90.1781363338388,-125.411996738862)) ;
#86296=UNCERTAINTY_MEASURE_WITH_UNIT(LENGTH_MEASURE(0.01),#86331,
'DISTANCE_ACCURACY_VALUE',
'Maximum model space distance between geometric entities at asserted c
onnectivities') ;
#86304=UNCERTAINTY_MEASURE_WITH_UNIT(LENGTH_MEASURE(0.01),#86331,
'DISTANCE_ACCURACY_VALUE',
'Maximum model space distance between geometric entities at asserted c
onnectivities') ;
#86322=(
GEOMETRIC_REPRESENTATION_CONTEXT(3)
GLOBAL_UNCERTAINTY_ASSIGNED_CONTEXT((#86296))
GLOBAL_UNIT_ASSIGNED_CONTEXT((#86331,#86333,#86334))
REPRESENTATION_CONTEXT('','3D')
) ;
#86330=(
GEOMETRIC_REPRESENTATION_CONTEXT(3)
GLOBAL_UNCERTAINTY_ASSIGNED_CONTEXT((#86304))
GLOBAL_UNIT_ASSIGNED_CONTEXT((#86331,#86333,#86334))
REPRESENTATION_CONTEXT('','3D')
) ;
#86331=(
LENGTH_UNIT()
NAMED_UNIT(*)
SI_UNIT(.MILLI.,.METRE.)
) ;
#86333=(
NAMED_UNIT(*)
PLANE_ANGLE_UNIT()
SI_UNIT($,.RADIAN.)
) ;
#86334=(
NAMED_UNIT(*)
SI_UNIT($,.STERADIAN.)
SOLID_ANGLE_UNIT()
) ;
#86352=SHAPE_DEFINITION_REPRESENTATION(#86423,#86468) ;
#86423=PRODUCT_DEFINITION_SHAPE('',$,#86494) ;
#86468=SHAPE_REPRESENTATION('',(#36343),#86322) ;
#86476=PRODUCT_DEFINITION_CONTEXT('part definition',#86553,'design') ;
#86494=PRODUCT_DEFINITION('Breadboard','Breadboard',#86519,#86476) ;
#86519=PRODUCT_DEFINITION_FORMATION('',$,#86572) ;
#86553=APPLICATION_CONTEXT(
'Core Data for Automotive Mechanical Design Process') ;
#86554=PRODUCT_CONTEXT('part definition',#86553,'mechanical') ;
#86572=PRODUCT('Breadboard','Breadboard',$,(#86554)) ;
#86584=PRESENTATION_STYLE_ASSIGNMENT((#86589)) ;
#86589=SURFACE_STYLE_USAGE(.BOTH.,#86594) ;
#86594=SURFACE_SIDE_STYLE('',(#86599)) ;
#86599=SURFACE_STYLE_FILL_AREA(#86604) ;
#86604=FILL_AREA_STYLE('Opaque(64,64,64)',(#86609)) ;
#86609=FILL_AREA_STYLE_COLOUR('Opaque(64,64,64)',#86614) ;
#86614=COLOUR_RGB('Opaque(64,64,64)', 0.31764706, 0.68627451, 0.89019608) ;
ENDSEC;
END-ISO-10303-21;
